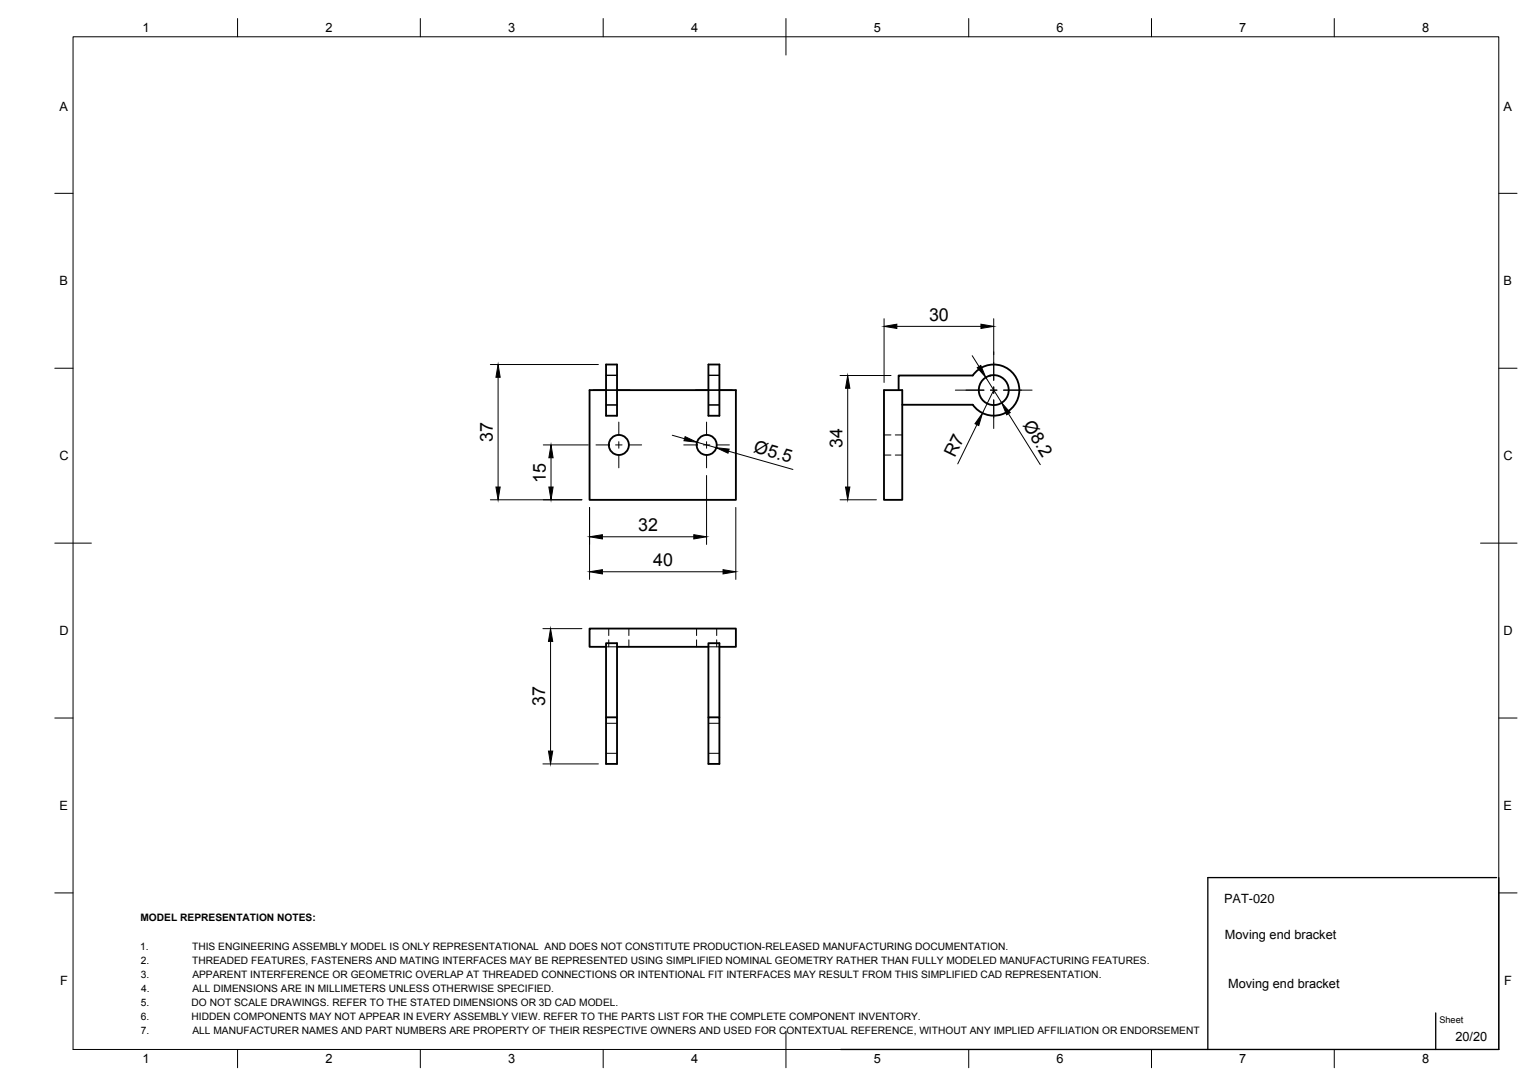
ISO-10303-21;
HEADER;
/* Generated by software containing ST-Developer
 * from STEP Tools, Inc. (www.steptools.com) 
 */

FILE_DESCRIPTION(
/* description */ ('Cable chain and bracket set'),
/* implementation_level */ '2;1');

FILE_NAME(
/* name */ 'Moving end bracket.step',
/* time_stamp */ '2026-10-29T17:19:47-07:00',
/* author */ (''),
/* organization */ (''),
/* preprocessor_version */ 'ST-DEVELOPER v20.2',
/* originating_system */ 'Autodesk Translation Framework v15.17.0.0',
/* authorisation */ '');

FILE_SCHEMA (('AUTOMOTIVE_DESIGN { 1 0 10303 214 3 1 1 }'));
ENDSEC;

DATA;
#10=MECHANICAL_DESIGN_GEOMETRIC_PRESENTATION_REPRESENTATION('',(#344),#5929);
#318=SHAPE_REPRESENTATION_RELATIONSHIP('SRR','None',#6055,#331);
#331=ADVANCED_BREP_SHAPE_REPRESENTATION('',(#357),#5922);
#344=STYLED_ITEM('',(#6199),#357);
#357=MANIFOLD_SOLID_BREP('Body1',#3338);
#385=FACE_BOUND('',#830,.T.);
#386=FACE_BOUND('',#833,.T.);
#387=FACE_BOUND('',#839,.T.);
#388=FACE_BOUND('',#842,.T.);
#389=FACE_BOUND('',#849,.T.);
#390=FACE_BOUND('',#850,.T.);
#391=FACE_BOUND('',#852,.T.);
#392=FACE_BOUND('',#853,.T.);
#467=PLANE('',#3619);
#468=PLANE('',#3620);
#469=PLANE('',#3621);
#470=PLANE('',#3622);
#471=PLANE('',#3623);
#472=PLANE('',#3624);
#473=PLANE('',#3628);
#474=PLANE('',#3629);
#475=PLANE('',#3630);
#476=PLANE('',#3631);
#477=PLANE('',#3632);
#478=PLANE('',#3633);
#479=PLANE('',#3634);
#480=PLANE('',#3635);
#481=PLANE('',#3636);
#482=PLANE('',#3637);
#620=FACE_OUTER_BOUND('',#824,.T.);
#621=FACE_OUTER_BOUND('',#825,.T.);
#622=FACE_OUTER_BOUND('',#826,.T.);
#623=FACE_OUTER_BOUND('',#827,.T.);
#624=FACE_OUTER_BOUND('',#828,.T.);
#625=FACE_OUTER_BOUND('',#829,.T.);
#626=FACE_OUTER_BOUND('',#831,.T.);
#627=FACE_OUTER_BOUND('',#832,.T.);
#628=FACE_OUTER_BOUND('',#834,.T.);
#629=FACE_OUTER_BOUND('',#835,.T.);
#630=FACE_OUTER_BOUND('',#836,.T.);
#631=FACE_OUTER_BOUND('',#837,.T.);
#632=FACE_OUTER_BOUND('',#838,.T.);
#633=FACE_OUTER_BOUND('',#840,.T.);
#634=FACE_OUTER_BOUND('',#841,.T.);
#635=FACE_OUTER_BOUND('',#843,.T.);
#636=FACE_OUTER_BOUND('',#844,.T.);
#637=FACE_OUTER_BOUND('',#845,.T.);
#638=FACE_OUTER_BOUND('',#846,.T.);
#639=FACE_OUTER_BOUND('',#847,.T.);
#640=FACE_OUTER_BOUND('',#848,.T.);
#641=FACE_OUTER_BOUND('',#851,.T.);
#824=EDGE_LOOP('',(#2679,#2680,#2681,#2682));
#825=EDGE_LOOP('',(#2683,#2684,#2685,#2686));
#826=EDGE_LOOP('',(#2687,#2688,#2689,#2690));
#827=EDGE_LOOP('',(#2691,#2692,#2693,#2694));
#828=EDGE_LOOP('',(#2695,#2696,#2697,#2698));
#829=EDGE_LOOP('',(#2699,#2700,#2701,#2702,#2703,#2704));
#830=EDGE_LOOP('',(#2705));
#831=EDGE_LOOP('',(#2706,#2707,#2708,#2709));
#832=EDGE_LOOP('',(#2710,#2711,#2712,#2713,#2714,#2715));
#833=EDGE_LOOP('',(#2716));
#834=EDGE_LOOP('',(#2717,#2718,#2719,#2720));
#835=EDGE_LOOP('',(#2721,#2722,#2723,#2724));
#836=EDGE_LOOP('',(#2725,#2726,#2727,#2728,#2729,#2730,#2731,#2732,#2733,
#2734,#2735,#2736));
#837=EDGE_LOOP('',(#2737,#2738,#2739,#2740));
#838=EDGE_LOOP('',(#2741,#2742,#2743,#2744,#2745,#2746));
#839=EDGE_LOOP('',(#2747));
#840=EDGE_LOOP('',(#2748,#2749,#2750,#2751));
#841=EDGE_LOOP('',(#2752,#2753,#2754,#2755,#2756,#2757));
#842=EDGE_LOOP('',(#2758));
#843=EDGE_LOOP('',(#2759,#2760,#2761,#2762));
#844=EDGE_LOOP('',(#2763,#2764,#2765,#2766));
#845=EDGE_LOOP('',(#2767,#2768,#2769,#2770));
#846=EDGE_LOOP('',(#2771,#2772,#2773,#2774));
#847=EDGE_LOOP('',(#2775,#2776,#2777,#2778));
#848=EDGE_LOOP('',(#2779,#2780,#2781,#2782,#2783,#2784,#2785,#2786,#2787,
#2788,#2789,#2790));
#849=EDGE_LOOP('',(#2791));
#850=EDGE_LOOP('',(#2792));
#851=EDGE_LOOP('',(#2793,#2794,#2795,#2796));
#852=EDGE_LOOP('',(#2797));
#853=EDGE_LOOP('',(#2798));
#1064=LINE('',#5363,#1324);
#1065=LINE('',#5369,#1325);
#1066=LINE('',#5375,#1326);
#1067=LINE('',#5381,#1327);
#1068=LINE('',#5386,#1328);
#1069=LINE('',#5390,#1329);
#1070=LINE('',#5394,#1330);
#1071=LINE('',#5396,#1331);
#1072=LINE('',#5398,#1332);
#1073=LINE('',#5400,#1333);
#1074=LINE('',#5401,#1334);
#1075=LINE('',#5404,#1335);
#1076=LINE('',#5405,#1336);
#1077=LINE('',#5408,#1337);
#1078=LINE('',#5410,#1338);
#1079=LINE('',#5412,#1339);
#1080=LINE('',#5413,#1340);
#1081=LINE('',#5415,#1341);
#1082=LINE('',#5417,#1342);
#1083=LINE('',#5420,#1343);
#1084=LINE('',#5422,#1344);
#1085=LINE('',#5424,#1345);
#1086=LINE('',#5426,#1346);
#1087=LINE('',#5428,#1347);
#1088=LINE('',#5430,#1348);
#1089=LINE('',#5432,#1349);
#1090=LINE('',#5434,#1350);
#1091=LINE('',#5435,#1351);
#1092=LINE('',#5439,#1352);
#1093=LINE('',#5443,#1353);
#1094=LINE('',#5447,#1354);
#1095=LINE('',#5448,#1355);
#1096=LINE('',#5450,#1356);
#1097=LINE('',#5451,#1357);
#1098=LINE('',#5454,#1358);
#1099=LINE('',#5455,#1359);
#1100=LINE('',#5458,#1360);
#1101=LINE('',#5459,#1361);
#1102=LINE('',#5460,#1362);
#1103=LINE('',#5462,#1363);
#1104=LINE('',#5466,#1364);
#1105=LINE('',#5468,#1365);
#1106=LINE('',#5469,#1366);
#1107=LINE('',#5472,#1367);
#1108=LINE('',#5474,#1368);
#1109=LINE('',#5475,#1369);
#1110=LINE('',#5477,#1370);
#1111=LINE('',#5478,#1371);
#1324=VECTOR('',#4313,0.274999999999999);
#1325=VECTOR('',#4320,0.274999999999999);
#1326=VECTOR('',#4327,0.41);
#1327=VECTOR('',#4334,0.41);
#1328=VECTOR('',#4339,1.);
#1329=VECTOR('',#4342,1.);
#1330=VECTOR('',#4347,1.);
#1331=VECTOR('',#4348,1.);
#1332=VECTOR('',#4349,1.);
#1333=VECTOR('',#4350,1.);
#1334=VECTOR('',#4351,1.);
#1335=VECTOR('',#4354,1.);
#1336=VECTOR('',#4355,1.);
#1337=VECTOR('',#4358,1.);
#1338=VECTOR('',#4359,1.);
#1339=VECTOR('',#4360,1.);
#1340=VECTOR('',#4361,1.);
#1341=VECTOR('',#4364,1.);
#1342=VECTOR('',#4367,1.);
#1343=VECTOR('',#4370,1.);
#1344=VECTOR('',#4371,1.);
#1345=VECTOR('',#4372,1.);
#1346=VECTOR('',#4373,1.);
#1347=VECTOR('',#4374,1.);
#1348=VECTOR('',#4375,1.);
#1349=VECTOR('',#4376,1.);
#1350=VECTOR('',#4377,1.);
#1351=VECTOR('',#4378,1.);
#1352=VECTOR('',#4381,1.);
#1353=VECTOR('',#4384,1.);
#1354=VECTOR('',#4389,1.);
#1355=VECTOR('',#4390,1.);
#1356=VECTOR('',#4391,1.);
#1357=VECTOR('',#4392,1.);
#1358=VECTOR('',#4395,1.);
#1359=VECTOR('',#4396,1.);
#1360=VECTOR('',#4399,1.);
#1361=VECTOR('',#4400,1.);
#1362=VECTOR('',#4401,1.);
#1363=VECTOR('',#4404,1.);
#1364=VECTOR('',#4409,1.);
#1365=VECTOR('',#4410,1.);
#1366=VECTOR('',#4411,1.);
#1367=VECTOR('',#4414,1.);
#1368=VECTOR('',#4415,1.);
#1369=VECTOR('',#4416,1.);
#1370=VECTOR('',#4419,1.);
#1371=VECTOR('',#4420,1.);
#1509=CIRCLE('',#3605,0.274999999999999);
#1510=CIRCLE('',#3606,0.274999999999999);
#1511=CIRCLE('',#3608,0.274999999999999);
#1512=CIRCLE('',#3609,0.274999999999999);
#1513=CIRCLE('',#3611,0.41);
#1514=CIRCLE('',#3612,0.41);
#1515=CIRCLE('',#3614,0.41);
#1516=CIRCLE('',#3615,0.41);
#1517=CIRCLE('',#3617,0.699999999999999);
#1518=CIRCLE('',#3618,0.699999999999999);
#1519=CIRCLE('',#3626,0.699999999999999);
#1520=CIRCLE('',#3627,0.699999999999999);
#1695=VERTEX_POINT('',#5360);
#1696=VERTEX_POINT('',#5362);
#1697=VERTEX_POINT('',#5366);
#1698=VERTEX_POINT('',#5368);
#1699=VERTEX_POINT('',#5372);
#1700=VERTEX_POINT('',#5374);
#1701=VERTEX_POINT('',#5378);
#1702=VERTEX_POINT('',#5380);
#1703=VERTEX_POINT('',#5384);
#1704=VERTEX_POINT('',#5385);
#1705=VERTEX_POINT('',#5387);
#1706=VERTEX_POINT('',#5389);
#1707=VERTEX_POINT('',#5393);
#1708=VERTEX_POINT('',#5395);
#1709=VERTEX_POINT('',#5397);
#1710=VERTEX_POINT('',#5399);
#1711=VERTEX_POINT('',#5403);
#1712=VERTEX_POINT('',#5407);
#1713=VERTEX_POINT('',#5409);
#1714=VERTEX_POINT('',#5411);
#1715=VERTEX_POINT('',#5419);
#1716=VERTEX_POINT('',#5421);
#1717=VERTEX_POINT('',#5423);
#1718=VERTEX_POINT('',#5425);
#1719=VERTEX_POINT('',#5427);
#1720=VERTEX_POINT('',#5429);
#1721=VERTEX_POINT('',#5431);
#1722=VERTEX_POINT('',#5433);
#1723=VERTEX_POINT('',#5437);
#1724=VERTEX_POINT('',#5438);
#1725=VERTEX_POINT('',#5440);
#1726=VERTEX_POINT('',#5442);
#1727=VERTEX_POINT('',#5446);
#1728=VERTEX_POINT('',#5449);
#1729=VERTEX_POINT('',#5453);
#1730=VERTEX_POINT('',#5457);
#1731=VERTEX_POINT('',#5465);
#1732=VERTEX_POINT('',#5467);
#1733=VERTEX_POINT('',#5471);
#1734=VERTEX_POINT('',#5473);
#2040=EDGE_CURVE('',#1695,#1695,#1509,.T.);
#2041=EDGE_CURVE('',#1695,#1696,#1064,.T.);
#2042=EDGE_CURVE('',#1696,#1696,#1510,.T.);
#2043=EDGE_CURVE('',#1697,#1697,#1511,.T.);
#2044=EDGE_CURVE('',#1697,#1698,#1065,.T.);
#2045=EDGE_CURVE('',#1698,#1698,#1512,.T.);
#2046=EDGE_CURVE('',#1699,#1699,#1513,.T.);
#2047=EDGE_CURVE('',#1699,#1700,#1066,.T.);
#2048=EDGE_CURVE('',#1700,#1700,#1514,.T.);
#2049=EDGE_CURVE('',#1701,#1701,#1515,.T.);
#2050=EDGE_CURVE('',#1701,#1702,#1067,.T.);
#2051=EDGE_CURVE('',#1702,#1702,#1516,.T.);
#2052=EDGE_CURVE('',#1703,#1704,#1068,.T.);
#2053=EDGE_CURVE('',#1703,#1705,#1517,.T.);
#2054=EDGE_CURVE('',#1706,#1705,#1069,.T.);
#2055=EDGE_CURVE('',#1704,#1706,#1518,.T.);
#2056=EDGE_CURVE('',#1706,#1707,#1070,.T.);
#2057=EDGE_CURVE('',#1708,#1707,#1071,.T.);
#2058=EDGE_CURVE('',#1709,#1708,#1072,.T.);
#2059=EDGE_CURVE('',#1709,#1710,#1073,.T.);
#2060=EDGE_CURVE('',#1710,#1704,#1074,.T.);
#2061=EDGE_CURVE('',#1711,#1705,#1075,.T.);
#2062=EDGE_CURVE('',#1707,#1711,#1076,.T.);
#2063=EDGE_CURVE('',#1703,#1712,#1077,.T.);
#2064=EDGE_CURVE('',#1712,#1713,#1078,.T.);
#2065=EDGE_CURVE('',#1714,#1713,#1079,.T.);
#2066=EDGE_CURVE('',#1711,#1714,#1080,.T.);
#2067=EDGE_CURVE('',#1712,#1710,#1081,.T.);
#2068=EDGE_CURVE('',#1713,#1709,#1082,.T.);
#2069=EDGE_CURVE('',#1715,#1708,#1083,.T.);
#2070=EDGE_CURVE('',#1716,#1715,#1084,.T.);
#2071=EDGE_CURVE('',#1716,#1717,#1085,.T.);
#2072=EDGE_CURVE('',#1717,#1718,#1086,.T.);
#2073=EDGE_CURVE('',#1719,#1718,#1087,.T.);
#2074=EDGE_CURVE('',#1719,#1720,#1088,.T.);
#2075=EDGE_CURVE('',#1720,#1721,#1089,.T.);
#2076=EDGE_CURVE('',#1721,#1722,#1090,.T.);
#2077=EDGE_CURVE('',#1714,#1722,#1091,.T.);
#2078=EDGE_CURVE('',#1723,#1724,#1092,.T.);
#2079=EDGE_CURVE('',#1723,#1725,#1519,.T.);
#2080=EDGE_CURVE('',#1726,#1725,#1093,.T.);
#2081=EDGE_CURVE('',#1724,#1726,#1520,.T.);
#2082=EDGE_CURVE('',#1726,#1727,#1094,.T.);
#2083=EDGE_CURVE('',#1722,#1727,#1095,.T.);
#2084=EDGE_CURVE('',#1721,#1728,#1096,.T.);
#2085=EDGE_CURVE('',#1728,#1724,#1097,.T.);
#2086=EDGE_CURVE('',#1729,#1725,#1098,.T.);
#2087=EDGE_CURVE('',#1727,#1729,#1099,.T.);
#2088=EDGE_CURVE('',#1723,#1730,#1100,.T.);
#2089=EDGE_CURVE('',#1730,#1720,#1101,.T.);
#2090=EDGE_CURVE('',#1729,#1719,#1102,.T.);
#2091=EDGE_CURVE('',#1730,#1728,#1103,.T.);
#2092=EDGE_CURVE('',#1731,#1716,#1104,.T.);
#2093=EDGE_CURVE('',#1732,#1715,#1105,.T.);
#2094=EDGE_CURVE('',#1731,#1732,#1106,.T.);
#2095=EDGE_CURVE('',#1733,#1731,#1107,.T.);
#2096=EDGE_CURVE('',#1734,#1732,#1108,.T.);
#2097=EDGE_CURVE('',#1733,#1734,#1109,.T.);
#2098=EDGE_CURVE('',#1717,#1733,#1110,.T.);
#2099=EDGE_CURVE('',#1718,#1734,#1111,.T.);
#2679=ORIENTED_EDGE('',*,*,#2040,.F.);
#2680=ORIENTED_EDGE('',*,*,#2041,.T.);
#2681=ORIENTED_EDGE('',*,*,#2042,.F.);
#2682=ORIENTED_EDGE('',*,*,#2041,.F.);
#2683=ORIENTED_EDGE('',*,*,#2043,.F.);
#2684=ORIENTED_EDGE('',*,*,#2044,.T.);
#2685=ORIENTED_EDGE('',*,*,#2045,.F.);
#2686=ORIENTED_EDGE('',*,*,#2044,.F.);
#2687=ORIENTED_EDGE('',*,*,#2046,.F.);
#2688=ORIENTED_EDGE('',*,*,#2047,.T.);
#2689=ORIENTED_EDGE('',*,*,#2048,.F.);
#2690=ORIENTED_EDGE('',*,*,#2047,.F.);
#2691=ORIENTED_EDGE('',*,*,#2049,.F.);
#2692=ORIENTED_EDGE('',*,*,#2050,.T.);
#2693=ORIENTED_EDGE('',*,*,#2051,.F.);
#2694=ORIENTED_EDGE('',*,*,#2050,.F.);
#2695=ORIENTED_EDGE('',*,*,#2052,.F.);
#2696=ORIENTED_EDGE('',*,*,#2053,.T.);
#2697=ORIENTED_EDGE('',*,*,#2054,.F.);
#2698=ORIENTED_EDGE('',*,*,#2055,.F.);
#2699=ORIENTED_EDGE('',*,*,#2055,.T.);
#2700=ORIENTED_EDGE('',*,*,#2056,.T.);
#2701=ORIENTED_EDGE('',*,*,#2057,.F.);
#2702=ORIENTED_EDGE('',*,*,#2058,.F.);
#2703=ORIENTED_EDGE('',*,*,#2059,.T.);
#2704=ORIENTED_EDGE('',*,*,#2060,.T.);
#2705=ORIENTED_EDGE('',*,*,#2051,.T.);
#2706=ORIENTED_EDGE('',*,*,#2054,.T.);
#2707=ORIENTED_EDGE('',*,*,#2061,.F.);
#2708=ORIENTED_EDGE('',*,*,#2062,.F.);
#2709=ORIENTED_EDGE('',*,*,#2056,.F.);
#2710=ORIENTED_EDGE('',*,*,#2063,.T.);
#2711=ORIENTED_EDGE('',*,*,#2064,.T.);
#2712=ORIENTED_EDGE('',*,*,#2065,.F.);
#2713=ORIENTED_EDGE('',*,*,#2066,.F.);
#2714=ORIENTED_EDGE('',*,*,#2061,.T.);
#2715=ORIENTED_EDGE('',*,*,#2053,.F.);
#2716=ORIENTED_EDGE('',*,*,#2049,.T.);
#2717=ORIENTED_EDGE('',*,*,#2052,.T.);
#2718=ORIENTED_EDGE('',*,*,#2060,.F.);
#2719=ORIENTED_EDGE('',*,*,#2067,.F.);
#2720=ORIENTED_EDGE('',*,*,#2063,.F.);
#2721=ORIENTED_EDGE('',*,*,#2068,.F.);
#2722=ORIENTED_EDGE('',*,*,#2064,.F.);
#2723=ORIENTED_EDGE('',*,*,#2067,.T.);
#2724=ORIENTED_EDGE('',*,*,#2059,.F.);
#2725=ORIENTED_EDGE('',*,*,#2065,.T.);
#2726=ORIENTED_EDGE('',*,*,#2068,.T.);
#2727=ORIENTED_EDGE('',*,*,#2058,.T.);
#2728=ORIENTED_EDGE('',*,*,#2069,.F.);
#2729=ORIENTED_EDGE('',*,*,#2070,.F.);
#2730=ORIENTED_EDGE('',*,*,#2071,.T.);
#2731=ORIENTED_EDGE('',*,*,#2072,.T.);
#2732=ORIENTED_EDGE('',*,*,#2073,.F.);
#2733=ORIENTED_EDGE('',*,*,#2074,.T.);
#2734=ORIENTED_EDGE('',*,*,#2075,.T.);
#2735=ORIENTED_EDGE('',*,*,#2076,.T.);
#2736=ORIENTED_EDGE('',*,*,#2077,.F.);
#2737=ORIENTED_EDGE('',*,*,#2078,.F.);
#2738=ORIENTED_EDGE('',*,*,#2079,.T.);
#2739=ORIENTED_EDGE('',*,*,#2080,.F.);
#2740=ORIENTED_EDGE('',*,*,#2081,.F.);
#2741=ORIENTED_EDGE('',*,*,#2081,.T.);
#2742=ORIENTED_EDGE('',*,*,#2082,.T.);
#2743=ORIENTED_EDGE('',*,*,#2083,.F.);
#2744=ORIENTED_EDGE('',*,*,#2076,.F.);
#2745=ORIENTED_EDGE('',*,*,#2084,.T.);
#2746=ORIENTED_EDGE('',*,*,#2085,.T.);
#2747=ORIENTED_EDGE('',*,*,#2048,.T.);
#2748=ORIENTED_EDGE('',*,*,#2080,.T.);
#2749=ORIENTED_EDGE('',*,*,#2086,.F.);
#2750=ORIENTED_EDGE('',*,*,#2087,.F.);
#2751=ORIENTED_EDGE('',*,*,#2082,.F.);
#2752=ORIENTED_EDGE('',*,*,#2088,.T.);
#2753=ORIENTED_EDGE('',*,*,#2089,.T.);
#2754=ORIENTED_EDGE('',*,*,#2074,.F.);
#2755=ORIENTED_EDGE('',*,*,#2090,.F.);
#2756=ORIENTED_EDGE('',*,*,#2086,.T.);
#2757=ORIENTED_EDGE('',*,*,#2079,.F.);
#2758=ORIENTED_EDGE('',*,*,#2046,.T.);
#2759=ORIENTED_EDGE('',*,*,#2078,.T.);
#2760=ORIENTED_EDGE('',*,*,#2085,.F.);
#2761=ORIENTED_EDGE('',*,*,#2091,.F.);
#2762=ORIENTED_EDGE('',*,*,#2088,.F.);
#2763=ORIENTED_EDGE('',*,*,#2075,.F.);
#2764=ORIENTED_EDGE('',*,*,#2089,.F.);
#2765=ORIENTED_EDGE('',*,*,#2091,.T.);
#2766=ORIENTED_EDGE('',*,*,#2084,.F.);
#2767=ORIENTED_EDGE('',*,*,#2092,.T.);
#2768=ORIENTED_EDGE('',*,*,#2070,.T.);
#2769=ORIENTED_EDGE('',*,*,#2093,.F.);
#2770=ORIENTED_EDGE('',*,*,#2094,.F.);
#2771=ORIENTED_EDGE('',*,*,#2095,.T.);
#2772=ORIENTED_EDGE('',*,*,#2094,.T.);
#2773=ORIENTED_EDGE('',*,*,#2096,.F.);
#2774=ORIENTED_EDGE('',*,*,#2097,.F.);
#2775=ORIENTED_EDGE('',*,*,#2098,.T.);
#2776=ORIENTED_EDGE('',*,*,#2097,.T.);
#2777=ORIENTED_EDGE('',*,*,#2099,.F.);
#2778=ORIENTED_EDGE('',*,*,#2072,.F.);
#2779=ORIENTED_EDGE('',*,*,#2066,.T.);
#2780=ORIENTED_EDGE('',*,*,#2077,.T.);
#2781=ORIENTED_EDGE('',*,*,#2083,.T.);
#2782=ORIENTED_EDGE('',*,*,#2087,.T.);
#2783=ORIENTED_EDGE('',*,*,#2090,.T.);
#2784=ORIENTED_EDGE('',*,*,#2073,.T.);
#2785=ORIENTED_EDGE('',*,*,#2099,.T.);
#2786=ORIENTED_EDGE('',*,*,#2096,.T.);
#2787=ORIENTED_EDGE('',*,*,#2093,.T.);
#2788=ORIENTED_EDGE('',*,*,#2069,.T.);
#2789=ORIENTED_EDGE('',*,*,#2057,.T.);
#2790=ORIENTED_EDGE('',*,*,#2062,.T.);
#2791=ORIENTED_EDGE('',*,*,#2042,.T.);
#2792=ORIENTED_EDGE('',*,*,#2045,.T.);
#2793=ORIENTED_EDGE('',*,*,#2071,.F.);
#2794=ORIENTED_EDGE('',*,*,#2092,.F.);
#2795=ORIENTED_EDGE('',*,*,#2095,.F.);
#2796=ORIENTED_EDGE('',*,*,#2098,.F.);
#2797=ORIENTED_EDGE('',*,*,#2040,.T.);
#2798=ORIENTED_EDGE('',*,*,#2043,.T.);
#3124=CYLINDRICAL_SURFACE('',#3604,0.274999999999999);
#3125=CYLINDRICAL_SURFACE('',#3607,0.274999999999999);
#3126=CYLINDRICAL_SURFACE('',#3610,0.41);
#3127=CYLINDRICAL_SURFACE('',#3613,0.41);
#3128=CYLINDRICAL_SURFACE('',#3616,0.699999999999999);
#3129=CYLINDRICAL_SURFACE('',#3625,0.699999999999999);
#3242=ADVANCED_FACE('',(#620),#3124,.F.);
#3243=ADVANCED_FACE('',(#621),#3125,.F.);
#3244=ADVANCED_FACE('',(#622),#3126,.F.);
#3245=ADVANCED_FACE('',(#623),#3127,.F.);
#3246=ADVANCED_FACE('',(#624),#3128,.T.);
#3247=ADVANCED_FACE('',(#625,#385),#467,.T.);
#3248=ADVANCED_FACE('',(#626),#468,.T.);
#3249=ADVANCED_FACE('',(#627,#386),#469,.F.);
#3250=ADVANCED_FACE('',(#628),#470,.T.);
#3251=ADVANCED_FACE('',(#629),#471,.T.);
#3252=ADVANCED_FACE('',(#630),#472,.T.);
#3253=ADVANCED_FACE('',(#631),#3129,.T.);
#3254=ADVANCED_FACE('',(#632,#387),#473,.T.);
#3255=ADVANCED_FACE('',(#633),#474,.T.);
#3256=ADVANCED_FACE('',(#634,#388),#475,.F.);
#3257=ADVANCED_FACE('',(#635),#476,.T.);
#3258=ADVANCED_FACE('',(#636),#477,.T.);
#3259=ADVANCED_FACE('',(#637),#478,.T.);
#3260=ADVANCED_FACE('',(#638),#479,.T.);
#3261=ADVANCED_FACE('',(#639),#480,.T.);
#3262=ADVANCED_FACE('',(#640,#389,#390),#481,.T.);
#3263=ADVANCED_FACE('',(#641,#391,#392),#482,.F.);
#3338=CLOSED_SHELL('',(#3242,#3243,#3244,#3245,#3246,#3247,#3248,#3249,
#3250,#3251,#3252,#3253,#3254,#3255,#3256,#3257,#3258,#3259,#3260,#3261,
#3262,#3263));
#3603=AXIS2_PLACEMENT_3D('',#5358,#4307,#4308);
#3604=AXIS2_PLACEMENT_3D('',#5359,#4309,#4310);
#3605=AXIS2_PLACEMENT_3D('',#5361,#4311,#4312);
#3606=AXIS2_PLACEMENT_3D('',#5364,#4314,#4315);
#3607=AXIS2_PLACEMENT_3D('',#5365,#4316,#4317);
#3608=AXIS2_PLACEMENT_3D('',#5367,#4318,#4319);
#3609=AXIS2_PLACEMENT_3D('',#5370,#4321,#4322);
#3610=AXIS2_PLACEMENT_3D('',#5371,#4323,#4324);
#3611=AXIS2_PLACEMENT_3D('',#5373,#4325,#4326);
#3612=AXIS2_PLACEMENT_3D('',#5376,#4328,#4329);
#3613=AXIS2_PLACEMENT_3D('',#5377,#4330,#4331);
#3614=AXIS2_PLACEMENT_3D('',#5379,#4332,#4333);
#3615=AXIS2_PLACEMENT_3D('',#5382,#4335,#4336);
#3616=AXIS2_PLACEMENT_3D('',#5383,#4337,#4338);
#3617=AXIS2_PLACEMENT_3D('',#5388,#4340,#4341);
#3618=AXIS2_PLACEMENT_3D('',#5391,#4343,#4344);
#3619=AXIS2_PLACEMENT_3D('',#5392,#4345,#4346);
#3620=AXIS2_PLACEMENT_3D('',#5402,#4352,#4353);
#3621=AXIS2_PLACEMENT_3D('',#5406,#4356,#4357);
#3622=AXIS2_PLACEMENT_3D('',#5414,#4362,#4363);
#3623=AXIS2_PLACEMENT_3D('',#5416,#4365,#4366);
#3624=AXIS2_PLACEMENT_3D('',#5418,#4368,#4369);
#3625=AXIS2_PLACEMENT_3D('',#5436,#4379,#4380);
#3626=AXIS2_PLACEMENT_3D('',#5441,#4382,#4383);
#3627=AXIS2_PLACEMENT_3D('',#5444,#4385,#4386);
#3628=AXIS2_PLACEMENT_3D('',#5445,#4387,#4388);
#3629=AXIS2_PLACEMENT_3D('',#5452,#4393,#4394);
#3630=AXIS2_PLACEMENT_3D('',#5456,#4397,#4398);
#3631=AXIS2_PLACEMENT_3D('',#5461,#4402,#4403);
#3632=AXIS2_PLACEMENT_3D('',#5463,#4405,#4406);
#3633=AXIS2_PLACEMENT_3D('',#5464,#4407,#4408);
#3634=AXIS2_PLACEMENT_3D('',#5470,#4412,#4413);
#3635=AXIS2_PLACEMENT_3D('',#5476,#4417,#4418);
#3636=AXIS2_PLACEMENT_3D('',#5479,#4421,#4422);
#3637=AXIS2_PLACEMENT_3D('',#5480,#4423,#4424);
#4307=DIRECTION('axis',(0.,0.,1.));
#4308=DIRECTION('refdir',(1.,0.,0.));
#4309=DIRECTION('center_axis',(0.,0.,1.));
#4310=DIRECTION('ref_axis',(1.,0.,0.));
#4311=DIRECTION('center_axis',(0.,0.,1.));
#4312=DIRECTION('ref_axis',(1.,0.,0.));
#4313=DIRECTION('',(0.,0.,1.));
#4314=DIRECTION('center_axis',(0.,0.,-1.));
#4315=DIRECTION('ref_axis',(1.,0.,0.));
#4316=DIRECTION('center_axis',(0.,0.,1.));
#4317=DIRECTION('ref_axis',(1.,0.,0.));
#4318=DIRECTION('center_axis',(0.,0.,1.));
#4319=DIRECTION('ref_axis',(1.,0.,0.));
#4320=DIRECTION('',(0.,0.,1.));
#4321=DIRECTION('center_axis',(0.,0.,-1.));
#4322=DIRECTION('ref_axis',(1.,0.,0.));
#4323=DIRECTION('center_axis',(0.,1.,0.));
#4324=DIRECTION('ref_axis',(1.,0.,0.));
#4325=DIRECTION('center_axis',(0.,1.,0.));
#4326=DIRECTION('ref_axis',(1.,0.,0.));
#4327=DIRECTION('',(0.,1.,0.));
#4328=DIRECTION('center_axis',(0.,-1.,0.));
#4329=DIRECTION('ref_axis',(1.,0.,0.));
#4330=DIRECTION('center_axis',(0.,1.,0.));
#4331=DIRECTION('ref_axis',(1.,0.,0.));
#4332=DIRECTION('center_axis',(0.,1.,0.));
#4333=DIRECTION('ref_axis',(1.,0.,0.));
#4334=DIRECTION('',(0.,1.,0.));
#4335=DIRECTION('center_axis',(0.,-1.,0.));
#4336=DIRECTION('ref_axis',(1.,0.,0.));
#4337=DIRECTION('center_axis',(0.,1.,0.));
#4338=DIRECTION('ref_axis',(-1.83697019872103E-16,0.,1.));
#4339=DIRECTION('',(0.,1.,0.));
#4340=DIRECTION('center_axis',(0.,1.,0.));
#4341=DIRECTION('ref_axis',(1.,0.,0.));
#4342=DIRECTION('',(0.,-1.,0.));
#4343=DIRECTION('center_axis',(0.,1.,0.));
#4344=DIRECTION('ref_axis',(1.,0.,0.));
#4345=DIRECTION('center_axis',(0.,1.,0.));
#4346=DIRECTION('ref_axis',(0.,0.,1.));
#4347=DIRECTION('',(0.,0.,-1.));
#4348=DIRECTION('',(1.,0.,0.));
#4349=DIRECTION('',(0.,0.,1.));
#4350=DIRECTION('',(-1.,0.,0.));
#4351=DIRECTION('',(0.,0.,1.));
#4352=DIRECTION('center_axis',(1.,0.,0.));
#4353=DIRECTION('ref_axis',(0.,0.,-1.));
#4354=DIRECTION('',(0.,0.,1.));
#4355=DIRECTION('',(0.,-1.,0.));
#4356=DIRECTION('center_axis',(0.,1.,0.));
#4357=DIRECTION('ref_axis',(1.,0.,0.));
#4358=DIRECTION('',(0.,0.,-1.));
#4359=DIRECTION('',(1.,0.,0.));
#4360=DIRECTION('',(0.,0.,-1.));
#4361=DIRECTION('',(-1.,0.,0.));
#4362=DIRECTION('center_axis',(-1.,0.,0.));
#4363=DIRECTION('ref_axis',(0.,0.,1.));
#4364=DIRECTION('',(0.,1.,0.));
#4365=DIRECTION('center_axis',(0.,0.,-1.));
#4366=DIRECTION('ref_axis',(-1.,0.,0.));
#4367=DIRECTION('',(0.,1.,0.));
#4368=DIRECTION('center_axis',(-1.,0.,0.));
#4369=DIRECTION('ref_axis',(0.,-1.,0.));
#4370=DIRECTION('',(0.,-1.,0.));
#4371=DIRECTION('',(0.,0.,1.));
#4372=DIRECTION('',(0.,-1.,0.));
#4373=DIRECTION('',(0.,0.,1.));
#4374=DIRECTION('',(0.,-1.,0.));
#4375=DIRECTION('',(0.,0.,-1.));
#4376=DIRECTION('',(0.,1.,0.));
#4377=DIRECTION('',(0.,0.,1.));
#4378=DIRECTION('',(0.,-1.,0.));
#4379=DIRECTION('center_axis',(0.,1.,0.));
#4380=DIRECTION('ref_axis',(-1.83697019872103E-16,0.,1.));
#4381=DIRECTION('',(0.,1.,0.));
#4382=DIRECTION('center_axis',(0.,1.,0.));
#4383=DIRECTION('ref_axis',(1.,0.,0.));
#4384=DIRECTION('',(0.,-1.,0.));
#4385=DIRECTION('center_axis',(0.,1.,0.));
#4386=DIRECTION('ref_axis',(1.,0.,0.));
#4387=DIRECTION('center_axis',(0.,1.,0.));
#4388=DIRECTION('ref_axis',(0.,0.,1.));
#4389=DIRECTION('',(0.,0.,-1.));
#4390=DIRECTION('',(1.,0.,0.));
#4391=DIRECTION('',(-1.,0.,0.));
#4392=DIRECTION('',(0.,0.,1.));
#4393=DIRECTION('center_axis',(1.,0.,0.));
#4394=DIRECTION('ref_axis',(0.,0.,-1.));
#4395=DIRECTION('',(0.,0.,1.));
#4396=DIRECTION('',(0.,-1.,0.));
#4397=DIRECTION('center_axis',(0.,1.,0.));
#4398=DIRECTION('ref_axis',(1.,0.,0.));
#4399=DIRECTION('',(0.,0.,-1.));
#4400=DIRECTION('',(1.,0.,0.));
#4401=DIRECTION('',(-1.,0.,0.));
#4402=DIRECTION('center_axis',(-1.,0.,0.));
#4403=DIRECTION('ref_axis',(0.,0.,1.));
#4404=DIRECTION('',(0.,1.,0.));
#4405=DIRECTION('center_axis',(0.,0.,-1.));
#4406=DIRECTION('ref_axis',(-1.,0.,0.));
#4407=DIRECTION('center_axis',(0.,1.,0.));
#4408=DIRECTION('ref_axis',(-1.,0.,0.));
#4409=DIRECTION('',(-1.,0.,0.));
#4410=DIRECTION('',(-1.,0.,0.));
#4411=DIRECTION('',(0.,0.,1.));
#4412=DIRECTION('center_axis',(1.,0.,0.));
#4413=DIRECTION('ref_axis',(0.,1.,0.));
#4414=DIRECTION('',(0.,1.,0.));
#4415=DIRECTION('',(0.,1.,0.));
#4416=DIRECTION('',(0.,0.,1.));
#4417=DIRECTION('center_axis',(0.,-1.,0.));
#4418=DIRECTION('ref_axis',(1.,0.,0.));
#4419=DIRECTION('',(1.,0.,0.));
#4420=DIRECTION('',(1.,0.,0.));
#4421=DIRECTION('center_axis',(0.,0.,1.));
#4422=DIRECTION('ref_axis',(1.,0.,0.));
#4423=DIRECTION('center_axis',(0.,0.,1.));
#4424=DIRECTION('ref_axis',(1.,0.,0.));
#5358=CARTESIAN_POINT('',(0.,0.,0.));
#5359=CARTESIAN_POINT('Origin',(21.5,-1.2,-0.1));
#5360=CARTESIAN_POINT('',(21.225,-1.2,0.));
#5361=CARTESIAN_POINT('Origin',(21.5,-1.2,0.));
#5362=CARTESIAN_POINT('',(21.225,-1.2,0.5));
#5363=CARTESIAN_POINT('',(21.225,-1.2,-0.1));
#5364=CARTESIAN_POINT('Origin',(21.5,-1.2,0.5));
#5365=CARTESIAN_POINT('Origin',(21.5,1.2,-0.1));
#5366=CARTESIAN_POINT('',(21.225,1.2,0.));
#5367=CARTESIAN_POINT('Origin',(21.5,1.2,0.));
#5368=CARTESIAN_POINT('',(21.225,1.2,0.5));
#5369=CARTESIAN_POINT('',(21.225,1.2,-0.1));
#5370=CARTESIAN_POINT('Origin',(21.5,1.2,0.5));
#5371=CARTESIAN_POINT('Origin',(20.,-1.7,3.));
#5372=CARTESIAN_POINT('',(19.59,-1.55,3.));
#5373=CARTESIAN_POINT('Origin',(20.,-1.55,3.));
#5374=CARTESIAN_POINT('',(19.59,-1.25,3.));
#5375=CARTESIAN_POINT('',(19.59,-1.7,3.));
#5376=CARTESIAN_POINT('Origin',(20.,-1.25,3.));
#5377=CARTESIAN_POINT('Origin',(20.,-1.7,3.));
#5378=CARTESIAN_POINT('',(19.59,1.25,3.));
#5379=CARTESIAN_POINT('Origin',(20.,1.25,3.));
#5380=CARTESIAN_POINT('',(19.59,1.55,3.));
#5381=CARTESIAN_POINT('',(19.59,-1.7,3.));
#5382=CARTESIAN_POINT('Origin',(20.,1.55,3.));
#5383=CARTESIAN_POINT('Origin',(20.,1.25,3.));
#5384=CARTESIAN_POINT('',(19.6,1.25,2.4255437353462));
#5385=CARTESIAN_POINT('',(19.6,1.55,2.4255437353462));
#5386=CARTESIAN_POINT('',(19.6,1.25,2.4255437353462));
#5387=CARTESIAN_POINT('',(20.4,1.25,2.4255437353462));
#5388=CARTESIAN_POINT('Origin',(20.,1.25,3.));
#5389=CARTESIAN_POINT('',(20.4,1.55,2.4255437353462));
#5390=CARTESIAN_POINT('',(20.4,1.25,2.4255437353462));
#5391=CARTESIAN_POINT('Origin',(20.,1.55,3.));
#5392=CARTESIAN_POINT('Origin',(20.,1.55,1.7));
#5393=CARTESIAN_POINT('',(20.4,1.55,0.5));
#5394=CARTESIAN_POINT('',(20.4,1.55,0.4));
#5395=CARTESIAN_POINT('',(20.,1.55,0.5));
#5396=CARTESIAN_POINT('',(20.75,1.55,0.5));
#5397=CARTESIAN_POINT('',(20.,1.55,0.4));
#5398=CARTESIAN_POINT('',(20.,1.55,0.85));
#5399=CARTESIAN_POINT('',(19.6,1.55,0.4));
#5400=CARTESIAN_POINT('',(19.6,1.55,0.4));
#5401=CARTESIAN_POINT('',(19.6,1.55,3.));
#5402=CARTESIAN_POINT('Origin',(20.4,1.25,3.));
#5403=CARTESIAN_POINT('',(20.4,1.25,0.5));
#5404=CARTESIAN_POINT('',(20.4,1.25,0.4));
#5405=CARTESIAN_POINT('',(20.4,0.625,0.5));
#5406=CARTESIAN_POINT('Origin',(20.,1.25,1.7));
#5407=CARTESIAN_POINT('',(19.6,1.25,0.4));
#5408=CARTESIAN_POINT('',(19.6,1.25,3.));
#5409=CARTESIAN_POINT('',(20.,1.25,0.4));
#5410=CARTESIAN_POINT('',(19.6,1.25,0.4));
#5411=CARTESIAN_POINT('',(20.,1.25,0.5));
#5412=CARTESIAN_POINT('',(20.,1.25,0.85));
#5413=CARTESIAN_POINT('',(20.75,1.25,0.5));
#5414=CARTESIAN_POINT('Origin',(19.6,1.25,0.4));
#5415=CARTESIAN_POINT('',(19.6,1.25,0.4));
#5416=CARTESIAN_POINT('Origin',(20.4,1.25,0.4));
#5417=CARTESIAN_POINT('',(20.,1.625,0.4));
#5418=CARTESIAN_POINT('Origin',(20.,2.,0.));
#5419=CARTESIAN_POINT('',(20.,2.,0.5));
#5420=CARTESIAN_POINT('',(20.,2.,0.5));
#5421=CARTESIAN_POINT('',(20.,2.,0.));
#5422=CARTESIAN_POINT('',(20.,2.,0.));
#5423=CARTESIAN_POINT('',(20.,-2.,0.));
#5424=CARTESIAN_POINT('',(20.,2.,0.));
#5425=CARTESIAN_POINT('',(20.,-2.,0.5));
#5426=CARTESIAN_POINT('',(20.,-2.,0.));
#5427=CARTESIAN_POINT('',(20.,-1.55,0.5));
#5428=CARTESIAN_POINT('',(20.,2.,0.5));
#5429=CARTESIAN_POINT('',(20.,-1.55,0.4));
#5430=CARTESIAN_POINT('',(20.,-1.55,0.85));
#5431=CARTESIAN_POINT('',(20.,-1.25,0.4));
#5432=CARTESIAN_POINT('',(20.,0.225,0.4));
#5433=CARTESIAN_POINT('',(20.,-1.25,0.5));
#5434=CARTESIAN_POINT('',(20.,-1.25,0.85));
#5435=CARTESIAN_POINT('',(20.,2.,0.5));
#5436=CARTESIAN_POINT('Origin',(20.,-1.55,3.));
#5437=CARTESIAN_POINT('',(19.6,-1.55,2.4255437353462));
#5438=CARTESIAN_POINT('',(19.6,-1.25,2.4255437353462));
#5439=CARTESIAN_POINT('',(19.6,-1.55,2.4255437353462));
#5440=CARTESIAN_POINT('',(20.4,-1.55,2.4255437353462));
#5441=CARTESIAN_POINT('Origin',(20.,-1.55,3.));
#5442=CARTESIAN_POINT('',(20.4,-1.25,2.4255437353462));
#5443=CARTESIAN_POINT('',(20.4,-1.55,2.4255437353462));
#5444=CARTESIAN_POINT('Origin',(20.,-1.25,3.));
#5445=CARTESIAN_POINT('Origin',(20.,-1.25,1.7));
#5446=CARTESIAN_POINT('',(20.4,-1.25,0.5));
#5447=CARTESIAN_POINT('',(20.4,-1.25,0.4));
#5448=CARTESIAN_POINT('',(20.75,-1.25,0.5));
#5449=CARTESIAN_POINT('',(19.6,-1.25,0.4));
#5450=CARTESIAN_POINT('',(19.6,-1.25,0.4));
#5451=CARTESIAN_POINT('',(19.6,-1.25,3.));
#5452=CARTESIAN_POINT('Origin',(20.4,-1.55,3.));
#5453=CARTESIAN_POINT('',(20.4,-1.55,0.5));
#5454=CARTESIAN_POINT('',(20.4,-1.55,0.4));
#5455=CARTESIAN_POINT('',(20.4,-0.775,0.5));
#5456=CARTESIAN_POINT('Origin',(20.,-1.55,1.7));
#5457=CARTESIAN_POINT('',(19.6,-1.55,0.4));
#5458=CARTESIAN_POINT('',(19.6,-1.55,3.));
#5459=CARTESIAN_POINT('',(19.6,-1.55,0.4));
#5460=CARTESIAN_POINT('',(20.75,-1.55,0.5));
#5461=CARTESIAN_POINT('Origin',(19.6,-1.55,0.4));
#5462=CARTESIAN_POINT('',(19.6,-1.55,0.4));
#5463=CARTESIAN_POINT('Origin',(20.4,-1.55,0.4));
#5464=CARTESIAN_POINT('Origin',(23.,2.,0.));
#5465=CARTESIAN_POINT('',(23.,2.,0.));
#5466=CARTESIAN_POINT('',(23.,2.,0.));
#5467=CARTESIAN_POINT('',(23.,2.,0.5));
#5468=CARTESIAN_POINT('',(23.,2.,0.5));
#5469=CARTESIAN_POINT('',(23.,2.,0.));
#5470=CARTESIAN_POINT('Origin',(23.,-2.,0.));
#5471=CARTESIAN_POINT('',(23.,-2.,0.));
#5472=CARTESIAN_POINT('',(23.,-2.,0.));
#5473=CARTESIAN_POINT('',(23.,-2.,0.5));
#5474=CARTESIAN_POINT('',(23.,-2.,0.5));
#5475=CARTESIAN_POINT('',(23.,-2.,0.));
#5476=CARTESIAN_POINT('Origin',(20.,-2.,0.));
#5477=CARTESIAN_POINT('',(20.,-2.,0.));
#5478=CARTESIAN_POINT('',(20.,-2.,0.5));
#5479=CARTESIAN_POINT('Origin',(21.5,0.,0.5));
#5480=CARTESIAN_POINT('Origin',(21.5,0.,0.));
#5898=UNCERTAINTY_MEASURE_WITH_UNIT(LENGTH_MEASURE(0.001),#5930,
'DISTANCE_ACCURACY_VALUE',
'Maximum model space distance between geometric entities at asserted c
onnectivities');
#5905=UNCERTAINTY_MEASURE_WITH_UNIT(LENGTH_MEASURE(0.001),#5930,
'DISTANCE_ACCURACY_VALUE',
'Maximum model space distance between geometric entities at asserted c
onnectivities');
#5922=(
GEOMETRIC_REPRESENTATION_CONTEXT(3)
GLOBAL_UNCERTAINTY_ASSIGNED_CONTEXT((#5898))
GLOBAL_UNIT_ASSIGNED_CONTEXT((#5930,#5932,#5933))
REPRESENTATION_CONTEXT('','3D')
);
#5929=(
GEOMETRIC_REPRESENTATION_CONTEXT(3)
GLOBAL_UNCERTAINTY_ASSIGNED_CONTEXT((#5905))
GLOBAL_UNIT_ASSIGNED_CONTEXT((#5930,#5932,#5933))
REPRESENTATION_CONTEXT('','3D')
);
#5930=(
LENGTH_UNIT()
NAMED_UNIT(*)
SI_UNIT(.CENTI.,.METRE.)
);
#5932=(
NAMED_UNIT(*)
PLANE_ANGLE_UNIT()
SI_UNIT($,.RADIAN.)
);
#5933=(
NAMED_UNIT(*)
SI_UNIT($,.STERADIAN.)
SOLID_ANGLE_UNIT()
);
#5950=SHAPE_DEFINITION_REPRESENTATION(#5979,#6055);
#5979=PRODUCT_DEFINITION_SHAPE('',$,#6079);
#6055=SHAPE_REPRESENTATION('',(#3603),#5922);
#6062=PRODUCT_DEFINITION_CONTEXT('part definition',#6133,'design');
#6079=PRODUCT_DEFINITION('Moving end bracket','Moving end bracket',#6102,
#6062);
#6102=PRODUCT_DEFINITION_FORMATION('',$,#6151);
#6133=APPLICATION_CONTEXT(
'Core Data for Automotive Mechanical Design Process');
#6134=PRODUCT_CONTEXT('part definition',#6133,'mechanical');
#6151=PRODUCT('Moving end bracket','Moving end bracket',
'Moving end bracket',(#6134));
#6193=COLOUR_RGB('Dark Blue',0.08,0.2,0.34);
#6194=FILL_AREA_STYLE_COLOUR('',#6193);
#6195=FILL_AREA_STYLE('',(#6194));
#6196=SURFACE_STYLE_FILL_AREA(#6195);
#6197=SURFACE_SIDE_STYLE('',(#6196));
#6198=SURFACE_STYLE_USAGE(.BOTH.,#6197);
#6199=PRESENTATION_STYLE_ASSIGNMENT((#6198));
ENDSEC;
END-ISO-10303-21;
